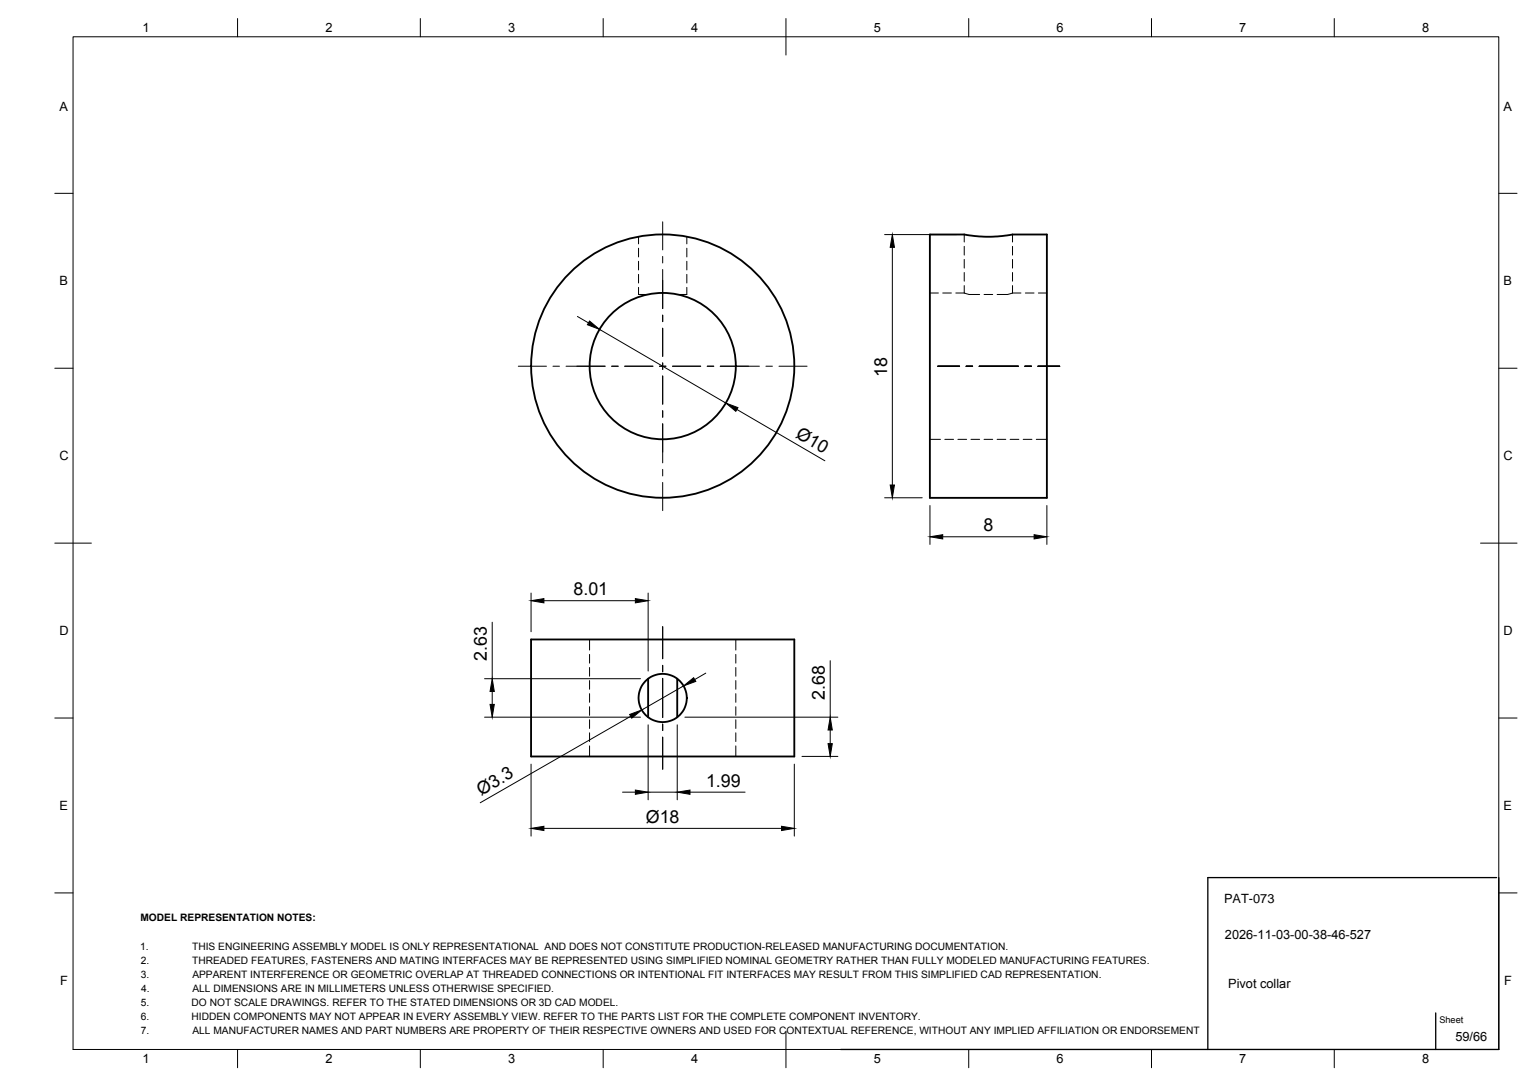
ISO-10303-21;
HEADER;
/* Generated by software containing ST-Developer
 * from STEP Tools, Inc. (www.steptools.com) 
 */

FILE_DESCRIPTION(
/* description */ ('Manual piston pump'),
/* implementation_level */ '2;1');

FILE_NAME(
/* name */ 'Pivot collar.step',
/* time_stamp */ '2026-11-02T16:54:23-08:00',
/* author */ (''),
/* organization */ (''),
/* preprocessor_version */ 'ST-DEVELOPER v20.2',
/* originating_system */ 'Autodesk Translation Framework v15.17.0.0',
/* authorisation */ '');

FILE_SCHEMA (('AUTOMOTIVE_DESIGN { 1 0 10303 214 3 1 1 }'));
ENDSEC;

DATA;
#10=MECHANICAL_DESIGN_GEOMETRIC_PRESENTATION_REPRESENTATION('',(#749),#19043);
#615=SHAPE_REPRESENTATION_RELATIONSHIP('SRR','None',#19365,#678);
#678=ADVANCED_BREP_SHAPE_REPRESENTATION('',(#817),#19032);
#749=STYLED_ITEM('',(#19661),#817);
#817=MANIFOLD_SOLID_BREP('Body1',#9537);
#1028=FACE_BOUND('',#2564,.T.);
#1029=FACE_BOUND('',#2566,.T.);
#1077=B_SPLINE_CURVE_WITH_KNOTS('',3,(#18383,#18384,#18385,#18386,#18387,
#18388),.UNSPECIFIED.,.F.,.F.,(4,2,4),(0.649292020015395,0.689320963667327,
0.7519713082482),.UNSPECIFIED.);
#1078=B_SPLINE_CURVE_WITH_KNOTS('',3,(#18392,#18393,#18394,#18395,#18396,
#18397),.UNSPECIFIED.,.F.,.F.,(4,2,4),(0.2506571027494,0.313307447330273,
0.353336390982205),.UNSPECIFIED.);
#1079=B_SPLINE_CURVE_WITH_KNOTS('',3,(#18398,#18399,#18400,#18401,#18402,
#18403),.UNSPECIFIED.,.F.,.F.,(4,2,4),(0.147977814516594,0.188006758168527,
0.2506571027494),.UNSPECIFIED.);
#1080=B_SPLINE_CURVE_WITH_KNOTS('',3,(#18404,#18405,#18406,#18407,#18408,
#18409),.UNSPECIFIED.,.F.,.F.,(4,2,4),(0.7519713082482,0.814621652829074,
0.854650596481005),.UNSPECIFIED.);
#1081=B_SPLINE_CURVE_WITH_KNOTS('',3,(#18413,#18414,#18415,#18416,#18417,
#18418,#18419,#18420,#18421,#18422),.UNSPECIFIED.,.F.,.F.,(4,2,2,2,4),(0.,
0.0623062782223143,0.124612556444629,0.186916384615149,0.249220212785669),
 .UNSPECIFIED.);
#1082=B_SPLINE_CURVE_WITH_KNOTS('',3,(#18424,#18425,#18426,#18427,#18428,
#18429,#18430,#18431,#18432,#18433),.UNSPECIFIED.,.F.,.F.,(4,2,2,2,4),(0.747660638357008,
0.809964466527528,0.872268294698049,0.934574572920363,0.996880851142677),
 .UNSPECIFIED.);
#1083=B_SPLINE_CURVE_WITH_KNOTS('',3,(#18434,#18435,#18436,#18437,#18438,
#18439,#18440,#18441,#18442,#18443,#18444,#18445,#18446,#18447,#18448,#18449,
#18450,#18451),.UNSPECIFIED.,.F.,.F.,(4,2,2,2,2,2,2,2,4),(0.249220212785669,
0.31152404095619,0.37382786912671,0.436134147349024,0.498440425571339,0.560746703793653,
0.623052982015967,0.685356810186488,0.747660638357008),.UNSPECIFIED.);
#1265=CYLINDRICAL_SURFACE('',#11312,0.165);
#1266=CYLINDRICAL_SURFACE('',#11315,0.5);
#1267=CYLINDRICAL_SURFACE('',#11318,0.9);
#1782=FACE_OUTER_BOUND('',#2558,.T.);
#1783=FACE_OUTER_BOUND('',#2559,.T.);
#1784=FACE_OUTER_BOUND('',#2560,.T.);
#1785=FACE_OUTER_BOUND('',#2561,.T.);
#1786=FACE_OUTER_BOUND('',#2562,.T.);
#1787=FACE_OUTER_BOUND('',#2563,.T.);
#1788=FACE_OUTER_BOUND('',#2565,.T.);
#2558=EDGE_LOOP('',(#8221,#8222));
#2559=EDGE_LOOP('',(#8223,#8224,#8225,#8226,#8227,#8228,#8229,#8230,#8231,
#8232,#8233));
#2560=EDGE_LOOP('',(#8234,#8235));
#2561=EDGE_LOOP('',(#8236,#8237,#8238,#8239,#8240,#8241,#8242,#8243,#8244,
#8245,#8246,#8247));
#2562=EDGE_LOOP('',(#8248,#8249,#8250,#8251,#8252,#8253,#8254,#8255,#8256));
#2563=EDGE_LOOP('',(#8257));
#2564=EDGE_LOOP('',(#8258));
#2565=EDGE_LOOP('',(#8259));
#2566=EDGE_LOOP('',(#8260));
#3088=CIRCLE('',#11311,0.165);
#3089=CIRCLE('',#11313,0.165);
#3090=CIRCLE('',#11316,0.5);
#3091=CIRCLE('',#11317,0.5);
#3092=CIRCLE('',#11319,0.9);
#3093=CIRCLE('',#11320,0.9);
#3648=LINE('',#18378,#4252);
#3649=LINE('',#18411,#4253);
#3650=LINE('',#18453,#4254);
#3651=LINE('',#18457,#4255);
#3652=LINE('',#18459,#4256);
#3653=LINE('',#18464,#4257);
#3654=LINE('',#18466,#4258);
#4252=VECTOR('',#14132,1.);
#4253=VECTOR('',#14139,0.165);
#4254=VECTOR('',#14142,1.);
#4255=VECTOR('',#14147,0.5);
#4256=VECTOR('',#14148,0.5);
#4257=VECTOR('',#14155,0.9);
#4258=VECTOR('',#14156,0.9);
#5008=VERTEX_POINT('',#18376);
#5009=VERTEX_POINT('',#18377);
#5010=VERTEX_POINT('',#18381);
#5011=VERTEX_POINT('',#18382);
#5012=VERTEX_POINT('',#18389);
#5013=VERTEX_POINT('',#18391);
#5014=VERTEX_POINT('',#18410);
#5015=VERTEX_POINT('',#18412);
#5016=VERTEX_POINT('',#18423);
#5017=VERTEX_POINT('',#18455);
#5018=VERTEX_POINT('',#18458);
#5019=VERTEX_POINT('',#18462);
#5020=VERTEX_POINT('',#18465);
#6097=EDGE_CURVE('',#5008,#5009,#3648,.T.);
#6098=EDGE_CURVE('',#5008,#5009,#3088,.T.);
#6099=EDGE_CURVE('',#5010,#5011,#1077,.T.);
#6100=EDGE_CURVE('',#5012,#5010,#3089,.T.);
#6101=EDGE_CURVE('',#5013,#5012,#1078,.T.);
#6102=EDGE_CURVE('',#5009,#5013,#1079,.T.);
#6103=EDGE_CURVE('',#5011,#5008,#1080,.T.);
#6104=EDGE_CURVE('',#5011,#5014,#3649,.T.);
#6105=EDGE_CURVE('',#5015,#5014,#1081,.T.);
#6106=EDGE_CURVE('',#5016,#5015,#1082,.T.);
#6107=EDGE_CURVE('',#5014,#5016,#1083,.T.);
#6108=EDGE_CURVE('',#5012,#5010,#3650,.T.);
#6109=EDGE_CURVE('',#5017,#5017,#3090,.T.);
#6110=EDGE_CURVE('',#5017,#5013,#3651,.T.);
#6111=EDGE_CURVE('',#5011,#5018,#3652,.T.);
#6112=EDGE_CURVE('',#5018,#5018,#3091,.T.);
#6113=EDGE_CURVE('',#5019,#5019,#3092,.T.);
#6114=EDGE_CURVE('',#5019,#5016,#3653,.T.);
#6115=EDGE_CURVE('',#5014,#5020,#3654,.T.);
#6116=EDGE_CURVE('',#5020,#5020,#3093,.T.);
#8221=ORIENTED_EDGE('',*,*,#6097,.F.);
#8222=ORIENTED_EDGE('',*,*,#6098,.T.);
#8223=ORIENTED_EDGE('',*,*,#6099,.F.);
#8224=ORIENTED_EDGE('',*,*,#6100,.F.);
#8225=ORIENTED_EDGE('',*,*,#6101,.F.);
#8226=ORIENTED_EDGE('',*,*,#6102,.F.);
#8227=ORIENTED_EDGE('',*,*,#6098,.F.);
#8228=ORIENTED_EDGE('',*,*,#6103,.F.);
#8229=ORIENTED_EDGE('',*,*,#6104,.T.);
#8230=ORIENTED_EDGE('',*,*,#6105,.F.);
#8231=ORIENTED_EDGE('',*,*,#6106,.F.);
#8232=ORIENTED_EDGE('',*,*,#6107,.F.);
#8233=ORIENTED_EDGE('',*,*,#6104,.F.);
#8234=ORIENTED_EDGE('',*,*,#6108,.F.);
#8235=ORIENTED_EDGE('',*,*,#6100,.T.);
#8236=ORIENTED_EDGE('',*,*,#6109,.F.);
#8237=ORIENTED_EDGE('',*,*,#6110,.T.);
#8238=ORIENTED_EDGE('',*,*,#6101,.T.);
#8239=ORIENTED_EDGE('',*,*,#6108,.T.);
#8240=ORIENTED_EDGE('',*,*,#6099,.T.);
#8241=ORIENTED_EDGE('',*,*,#6111,.T.);
#8242=ORIENTED_EDGE('',*,*,#6112,.T.);
#8243=ORIENTED_EDGE('',*,*,#6111,.F.);
#8244=ORIENTED_EDGE('',*,*,#6103,.T.);
#8245=ORIENTED_EDGE('',*,*,#6097,.T.);
#8246=ORIENTED_EDGE('',*,*,#6102,.T.);
#8247=ORIENTED_EDGE('',*,*,#6110,.F.);
#8248=ORIENTED_EDGE('',*,*,#6113,.F.);
#8249=ORIENTED_EDGE('',*,*,#6114,.T.);
#8250=ORIENTED_EDGE('',*,*,#6106,.T.);
#8251=ORIENTED_EDGE('',*,*,#6105,.T.);
#8252=ORIENTED_EDGE('',*,*,#6115,.T.);
#8253=ORIENTED_EDGE('',*,*,#6116,.T.);
#8254=ORIENTED_EDGE('',*,*,#6115,.F.);
#8255=ORIENTED_EDGE('',*,*,#6107,.T.);
#8256=ORIENTED_EDGE('',*,*,#6114,.F.);
#8257=ORIENTED_EDGE('',*,*,#6113,.T.);
#8258=ORIENTED_EDGE('',*,*,#6109,.T.);
#8259=ORIENTED_EDGE('',*,*,#6116,.F.);
#8260=ORIENTED_EDGE('',*,*,#6112,.F.);
#8844=PLANE('',#11310);
#8845=PLANE('',#11314);
#8846=PLANE('',#11321);
#8847=PLANE('',#11322);
#9387=ADVANCED_FACE('',(#1782),#8844,.T.);
#9388=ADVANCED_FACE('',(#1783),#1265,.F.);
#9389=ADVANCED_FACE('',(#1784),#8845,.T.);
#9390=ADVANCED_FACE('',(#1785),#1266,.F.);
#9391=ADVANCED_FACE('',(#1786),#1267,.T.);
#9392=ADVANCED_FACE('',(#1787,#1028),#8846,.T.);
#9393=ADVANCED_FACE('',(#1788,#1029),#8847,.F.);
#9537=CLOSED_SHELL('',(#9387,#9388,#9389,#9390,#9391,#9392,#9393));
#11309=AXIS2_PLACEMENT_3D('',#18374,#14128,#14129);
#11310=AXIS2_PLACEMENT_3D('',#18375,#14130,#14131);
#11311=AXIS2_PLACEMENT_3D('',#18379,#14133,#14134);
#11312=AXIS2_PLACEMENT_3D('',#18380,#14135,#14136);
#11313=AXIS2_PLACEMENT_3D('',#18390,#14137,#14138);
#11314=AXIS2_PLACEMENT_3D('',#18452,#14140,#14141);
#11315=AXIS2_PLACEMENT_3D('',#18454,#14143,#14144);
#11316=AXIS2_PLACEMENT_3D('',#18456,#14145,#14146);
#11317=AXIS2_PLACEMENT_3D('',#18460,#14149,#14150);
#11318=AXIS2_PLACEMENT_3D('',#18461,#14151,#14152);
#11319=AXIS2_PLACEMENT_3D('',#18463,#14153,#14154);
#11320=AXIS2_PLACEMENT_3D('',#18467,#14157,#14158);
#11321=AXIS2_PLACEMENT_3D('',#18468,#14159,#14160);
#11322=AXIS2_PLACEMENT_3D('',#18469,#14161,#14162);
#14128=DIRECTION('axis',(0.,0.,1.));
#14129=DIRECTION('refdir',(1.,0.,0.));
#14130=DIRECTION('center_axis',(0.,0.,1.));
#14131=DIRECTION('ref_axis',(1.,0.,0.));
#14132=DIRECTION('',(1.,0.,0.));
#14133=DIRECTION('center_axis',(0.,0.,1.));
#14134=DIRECTION('ref_axis',(1.,0.,0.));
#14135=DIRECTION('center_axis',(0.,0.,1.));
#14136=DIRECTION('ref_axis',(1.,0.,0.));
#14137=DIRECTION('center_axis',(0.,0.,1.));
#14138=DIRECTION('ref_axis',(1.,0.,0.));
#14139=DIRECTION('',(0.,0.,1.));
#14140=DIRECTION('center_axis',(0.,0.,1.));
#14141=DIRECTION('ref_axis',(1.,0.,0.));
#14142=DIRECTION('',(-1.,0.,0.));
#14143=DIRECTION('center_axis',(1.,0.,0.));
#14144=DIRECTION('ref_axis',(0.,0.,-1.));
#14145=DIRECTION('center_axis',(-1.,0.,0.));
#14146=DIRECTION('ref_axis',(0.,0.,-1.));
#14147=DIRECTION('',(-1.,0.,0.));
#14148=DIRECTION('',(-1.,0.,0.));
#14149=DIRECTION('center_axis',(-1.,0.,0.));
#14150=DIRECTION('ref_axis',(0.,0.,-1.));
#14151=DIRECTION('center_axis',(1.,0.,0.));
#14152=DIRECTION('ref_axis',(0.,0.,-1.));
#14153=DIRECTION('center_axis',(1.,0.,0.));
#14154=DIRECTION('ref_axis',(0.,0.,-1.));
#14155=DIRECTION('',(-1.,0.,0.));
#14156=DIRECTION('',(-1.,0.,0.));
#14157=DIRECTION('center_axis',(1.,0.,0.));
#14158=DIRECTION('ref_axis',(0.,0.,-1.));
#14159=DIRECTION('center_axis',(1.,0.,0.));
#14160=DIRECTION('ref_axis',(0.,0.,-1.));
#14161=DIRECTION('center_axis',(1.,0.,0.));
#14162=DIRECTION('ref_axis',(0.,0.,-1.));
#18374=CARTESIAN_POINT('',(0.,0.,0.));
#18375=CARTESIAN_POINT('Origin',(-3.6,-4.,10.49));
#18376=CARTESIAN_POINT('',(-3.73162446581089,-4.09949874371065,10.49));
#18377=CARTESIAN_POINT('',(-3.46837553418911,-4.09949874371065,10.49));
#18378=CARTESIAN_POINT('',(-4.,-4.09949874371065,10.49));
#18379=CARTESIAN_POINT('Origin',(-3.6,-4.,10.49));
#18380=CARTESIAN_POINT('Origin',(-3.6,-4.,10.49));
#18381=CARTESIAN_POINT('',(-3.73162446581089,-3.90050125628935,10.49));
#18382=CARTESIAN_POINT('',(-3.765,-4.,10.5));
#18383=CARTESIAN_POINT('Ctrl Pts',(-3.73162446581089,-3.90050125628935,
10.49));
#18384=CARTESIAN_POINT('Ctrl Pts',(-3.73987629702585,-3.91141740291719,
10.4922166181135));
#18385=CARTESIAN_POINT('Ctrl Pts',(-3.74695509902511,-3.92366776278637,
10.4943120869024));
#18386=CARTESIAN_POINT('Ctrl Pts',(-3.76079459046636,-3.95694557235505,
10.4985632587304));
#18387=CARTESIAN_POINT('Ctrl Pts',(-3.765,-3.97911655180638,10.5));
#18388=CARTESIAN_POINT('Ctrl Pts',(-3.765,-4.,10.5));
#18389=CARTESIAN_POINT('',(-3.46837553418911,-3.90050125628935,10.49));
#18390=CARTESIAN_POINT('Origin',(-3.6,-4.,10.49));
#18391=CARTESIAN_POINT('',(-3.435,-4.,10.5));
#18392=CARTESIAN_POINT('Ctrl Pts',(-3.435,-4.,10.5));
#18393=CARTESIAN_POINT('Ctrl Pts',(-3.435,-3.97911655180638,10.5));
#18394=CARTESIAN_POINT('Ctrl Pts',(-3.43920540953364,-3.95694557235505,
10.4985632587304));
#18395=CARTESIAN_POINT('Ctrl Pts',(-3.45304490097489,-3.92366776278637,
10.4943120869024));
#18396=CARTESIAN_POINT('Ctrl Pts',(-3.46012370297415,-3.91141740291719,
10.4922166181135));
#18397=CARTESIAN_POINT('Ctrl Pts',(-3.46837553418911,-3.90050125628935,
10.49));
#18398=CARTESIAN_POINT('Ctrl Pts',(-3.46837553418911,-4.09949874371065,
10.49));
#18399=CARTESIAN_POINT('Ctrl Pts',(-3.46012370297415,-4.08858259708281,
10.4922166181135));
#18400=CARTESIAN_POINT('Ctrl Pts',(-3.45304490097489,-4.07633223721363,
10.4943120869024));
#18401=CARTESIAN_POINT('Ctrl Pts',(-3.43920540953364,-4.04305442764495,
10.4985632587304));
#18402=CARTESIAN_POINT('Ctrl Pts',(-3.435,-4.02088344819362,10.5));
#18403=CARTESIAN_POINT('Ctrl Pts',(-3.435,-4.,10.5));
#18404=CARTESIAN_POINT('Ctrl Pts',(-3.765,-4.,10.5));
#18405=CARTESIAN_POINT('Ctrl Pts',(-3.765,-4.02088344819362,10.5));
#18406=CARTESIAN_POINT('Ctrl Pts',(-3.76079459046636,-4.04305442764495,
10.4985632587304));
#18407=CARTESIAN_POINT('Ctrl Pts',(-3.74695509902511,-4.07633223721363,
10.4943120869024));
#18408=CARTESIAN_POINT('Ctrl Pts',(-3.73987629702585,-4.08858259708281,
10.4922166181135));
#18409=CARTESIAN_POINT('Ctrl Pts',(-3.73162446581089,-4.09949874371065,
10.49));
#18410=CARTESIAN_POINT('',(-3.765,-4.,10.9));
#18411=CARTESIAN_POINT('',(-3.765,-4.,10.49));
#18412=CARTESIAN_POINT('',(-3.6,-4.165,10.8847457261835));
#18413=CARTESIAN_POINT('Ctrl Pts',(-3.6,-4.165,10.8847457261835));
#18414=CARTESIAN_POINT('Ctrl Pts',(-3.62076875940744,-4.165,10.8847457261835));
#18415=CARTESIAN_POINT('Ctrl Pts',(-3.64288889507334,-4.16083971900758,
10.8855527595053));
#18416=CARTESIAN_POINT('Ctrl Pts',(-3.68352706263377,-4.14398647021669,
10.88844864815));
#18417=CARTESIAN_POINT('Ctrl Pts',(-3.70204924397737,-4.13129599381419,
10.8904936048516));
#18418=CARTESIAN_POINT('Ctrl Pts',(-3.73129541878344,-4.10204981900812,
10.8943172343239));
#18419=CARTESIAN_POINT('Ctrl Pts',(-3.74398634598358,-4.08352739209068,
10.8963470888995));
#18420=CARTESIAN_POINT('Ctrl Pts',(-3.76083992183864,-4.04288837609341,
10.8992082718606));
#18421=CARTESIAN_POINT('Ctrl Pts',(-3.765,-4.02076794272351,10.9));
#18422=CARTESIAN_POINT('Ctrl Pts',(-3.765,-4.,10.9));
#18423=CARTESIAN_POINT('',(-3.435,-4.,10.9));
#18424=CARTESIAN_POINT('Ctrl Pts',(-3.435,-4.,10.9));
#18425=CARTESIAN_POINT('Ctrl Pts',(-3.435,-4.02076794272351,10.9));
#18426=CARTESIAN_POINT('Ctrl Pts',(-3.43916007816136,-4.04288837609341,
10.8992082718606));
#18427=CARTESIAN_POINT('Ctrl Pts',(-3.45601365401642,-4.08352739209068,
10.8963470888995));
#18428=CARTESIAN_POINT('Ctrl Pts',(-3.46870458121656,-4.10204981900812,
10.8943172343239));
#18429=CARTESIAN_POINT('Ctrl Pts',(-3.49795075602263,-4.13129599381419,
10.8904936048516));
#18430=CARTESIAN_POINT('Ctrl Pts',(-3.51647293736623,-4.14398647021669,
10.88844864815));
#18431=CARTESIAN_POINT('Ctrl Pts',(-3.55711110492666,-4.16083971900758,
10.8855527595053));
#18432=CARTESIAN_POINT('Ctrl Pts',(-3.57923124059256,-4.165,10.8847457261835));
#18433=CARTESIAN_POINT('Ctrl Pts',(-3.6,-4.165,10.8847457261835));
#18434=CARTESIAN_POINT('Ctrl Pts',(-3.765,-4.,10.9));
#18435=CARTESIAN_POINT('Ctrl Pts',(-3.765,-3.97923205727649,10.9));
#18436=CARTESIAN_POINT('Ctrl Pts',(-3.76083992183864,-3.95711162390659,
10.8992082718606));
#18437=CARTESIAN_POINT('Ctrl Pts',(-3.74398634598358,-3.91647260790932,
10.8963470888995));
#18438=CARTESIAN_POINT('Ctrl Pts',(-3.73129541878344,-3.89795018099187,
10.8943172343239));
#18439=CARTESIAN_POINT('Ctrl Pts',(-3.70204924397737,-3.86870400618581,
10.8904936048516));
#18440=CARTESIAN_POINT('Ctrl Pts',(-3.68352706263377,-3.85601352978331,
10.88844864815));
#18441=CARTESIAN_POINT('Ctrl Pts',(-3.64288889507334,-3.83916028099242,
10.8855527595053));
#18442=CARTESIAN_POINT('Ctrl Pts',(-3.62076875940744,-3.835,10.8847457261835));
#18443=CARTESIAN_POINT('Ctrl Pts',(-3.57923124059256,-3.835,10.8847457261835));
#18444=CARTESIAN_POINT('Ctrl Pts',(-3.55711110492665,-3.83916028099242,
10.8855527595053));
#18445=CARTESIAN_POINT('Ctrl Pts',(-3.51647293736623,-3.85601352978331,
10.88844864815));
#18446=CARTESIAN_POINT('Ctrl Pts',(-3.49795075602263,-3.86870400618581,
10.8904936048516));
#18447=CARTESIAN_POINT('Ctrl Pts',(-3.46870458121656,-3.89795018099187,
10.8943172343239));
#18448=CARTESIAN_POINT('Ctrl Pts',(-3.45601365401642,-3.91647260790932,
10.8963470888995));
#18449=CARTESIAN_POINT('Ctrl Pts',(-3.43916007816136,-3.95711162390659,
10.8992082718606));
#18450=CARTESIAN_POINT('Ctrl Pts',(-3.435,-3.97923205727649,10.9));
#18451=CARTESIAN_POINT('Ctrl Pts',(-3.435,-4.,10.9));
#18452=CARTESIAN_POINT('Origin',(-3.6,-4.,10.49));
#18453=CARTESIAN_POINT('',(-4.,-3.90050125628935,10.49));
#18454=CARTESIAN_POINT('Origin',(-4.,-4.,10.));
#18455=CARTESIAN_POINT('',(-3.2,-4.,10.5));
#18456=CARTESIAN_POINT('Origin',(-3.2,-4.,10.));
#18457=CARTESIAN_POINT('',(-4.,-4.,10.5));
#18458=CARTESIAN_POINT('',(-4.,-4.,10.5));
#18459=CARTESIAN_POINT('',(-4.,-4.,10.5));
#18460=CARTESIAN_POINT('Origin',(-4.,-4.,10.));
#18461=CARTESIAN_POINT('Origin',(-4.,-4.,10.));
#18462=CARTESIAN_POINT('',(-3.2,-4.,10.9));
#18463=CARTESIAN_POINT('Origin',(-3.2,-4.,10.));
#18464=CARTESIAN_POINT('',(-4.,-4.,10.9));
#18465=CARTESIAN_POINT('',(-4.,-4.,10.9));
#18466=CARTESIAN_POINT('',(-4.,-4.,10.9));
#18467=CARTESIAN_POINT('Origin',(-4.,-4.,10.));
#18468=CARTESIAN_POINT('Origin',(-3.2,-4.,10.));
#18469=CARTESIAN_POINT('Origin',(-4.,-4.,10.));
#18961=UNCERTAINTY_MEASURE_WITH_UNIT(LENGTH_MEASURE(0.001),#19044,
'DISTANCE_ACCURACY_VALUE',
'Maximum model space distance between geometric entities at asserted c
onnectivities');
#18972=UNCERTAINTY_MEASURE_WITH_UNIT(LENGTH_MEASURE(0.001),#19044,
'DISTANCE_ACCURACY_VALUE',
'Maximum model space distance between geometric entities at asserted c
onnectivities');
#19032=(
GEOMETRIC_REPRESENTATION_CONTEXT(3)
GLOBAL_UNCERTAINTY_ASSIGNED_CONTEXT((#18961))
GLOBAL_UNIT_ASSIGNED_CONTEXT((#19044,#19046,#19047))
REPRESENTATION_CONTEXT('','3D')
);
#19043=(
GEOMETRIC_REPRESENTATION_CONTEXT(3)
GLOBAL_UNCERTAINTY_ASSIGNED_CONTEXT((#18972))
GLOBAL_UNIT_ASSIGNED_CONTEXT((#19044,#19046,#19047))
REPRESENTATION_CONTEXT('','3D')
);
#19044=(
LENGTH_UNIT()
NAMED_UNIT(*)
SI_UNIT(.CENTI.,.METRE.)
);
#19046=(
NAMED_UNIT(*)
PLANE_ANGLE_UNIT()
SI_UNIT($,.RADIAN.)
);
#19047=(
NAMED_UNIT(*)
SI_UNIT($,.STERADIAN.)
SOLID_ANGLE_UNIT()
);
#19107=SHAPE_DEFINITION_REPRESENTATION(#19264,#19365);
#19264=PRODUCT_DEFINITION_SHAPE('',$,#19436);
#19365=SHAPE_REPRESENTATION('',(#11309),#19032);
#19376=PRODUCT_DEFINITION_CONTEXT('part definition',#19588,'design');
#19436=PRODUCT_DEFINITION('2026-11-03-00-38-46-527','Pivot collar',#19506,
#19376);
#19506=PRODUCT_DEFINITION_FORMATION('',$,#19649);
#19588=APPLICATION_CONTEXT(
'Core Data for Automotive Mechanical Design Process');
#19589=PRODUCT_CONTEXT('part definition',#19588,'mechanical');
#19649=PRODUCT('2026-11-03-00-38-46-527','Pivot collar','Pivot collar',
(#19589));
#19661=PRESENTATION_STYLE_ASSIGNMENT((#19667));
#19667=SURFACE_STYLE_USAGE(.BOTH.,#19673);
#19673=SURFACE_SIDE_STYLE('',(#19679));
#19679=SURFACE_STYLE_FILL_AREA(#19685);
#19685=FILL_AREA_STYLE('CAD Library Painted - Engineering blue',(#19691));
#19691=FILL_AREA_STYLE_COLOUR('CAD Library Painted - Engineering blue',
#19697);
#19697=COLOUR_RGB('CAD Library Painted - Engineering blue',0.12156862745098,
0.356862745098039,0.6);
ENDSEC;
END-ISO-10303-21;
